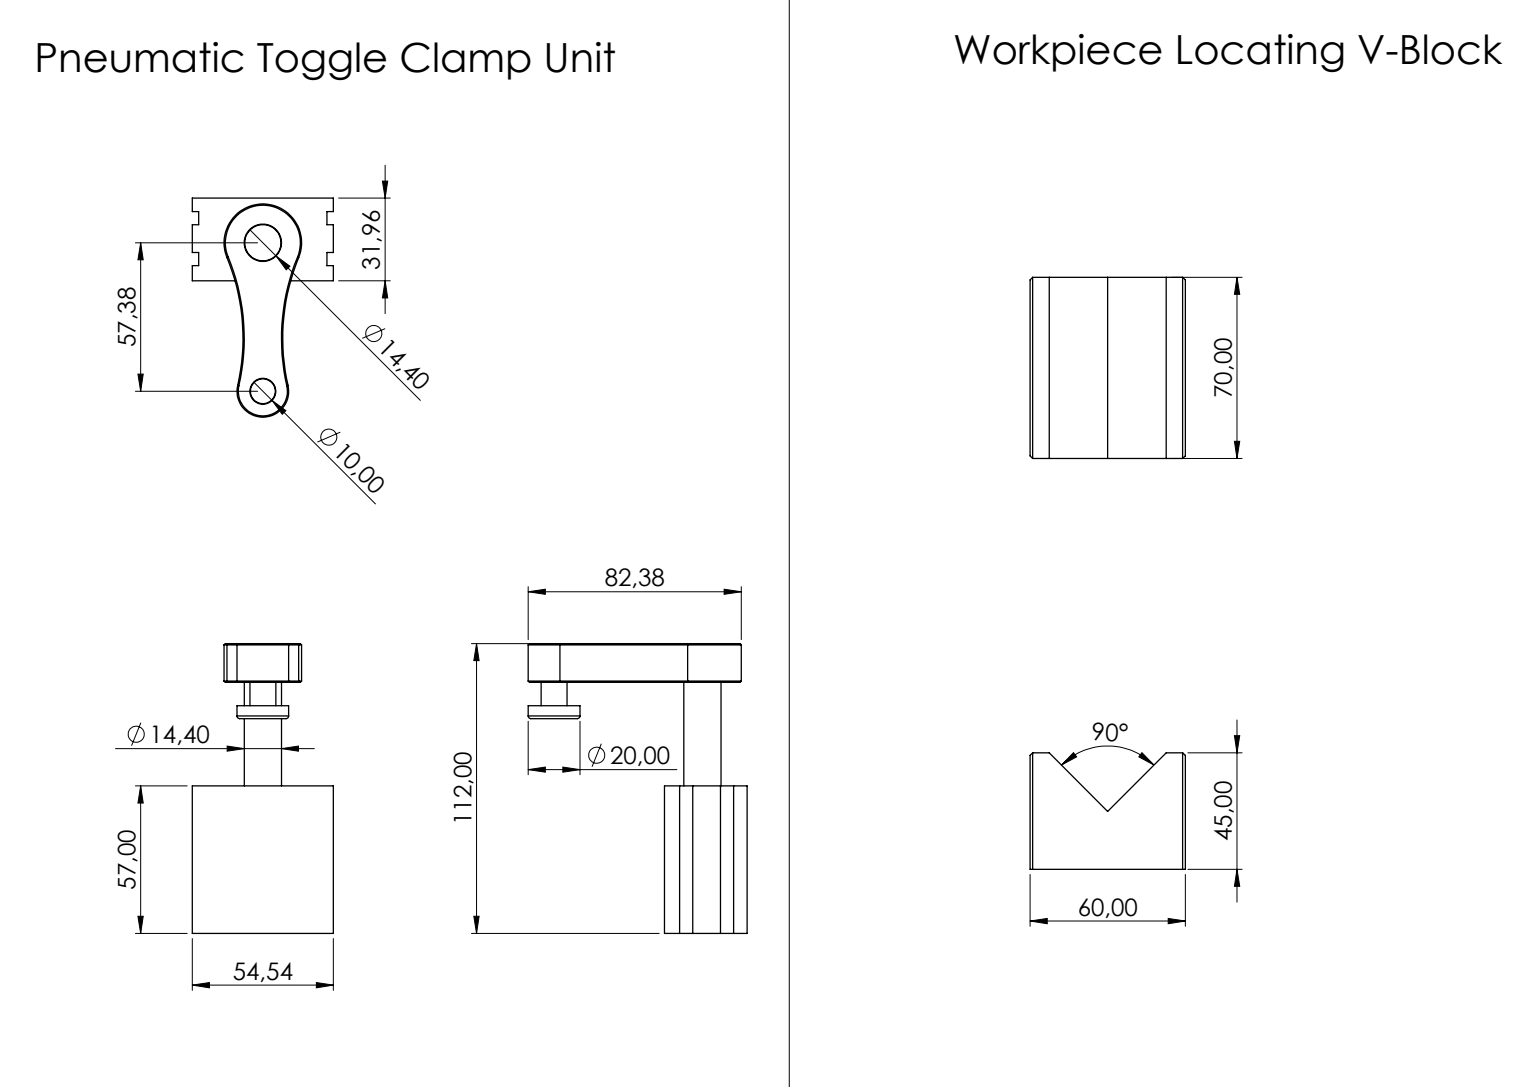
ISO-10303-21;
HEADER;
FILE_DESCRIPTION (('STEP AP214'),
    '1' );
FILE_NAME ('Workpiece Locating V-Block.step',
    '2026-10-07T11:37:37',
    ( '' ),
    ( '' ),
    'SwSTEP 2.0',
    'SolidWorks 2020',
    '' );
FILE_SCHEMA (( 'AUTOMOTIVE_DESIGN' ));
ENDSEC;

DATA;
#31=VECTOR ( 'NONE', #9113, 1000.000000000000000 ) ;
#48=LINE ( 'NONE', #40482, #73685 ) ;
#312=CARTESIAN_POINT ( 'NONE',  ( 29.00000000000003553, 172.0000000000000000, 183.8826257785461280 ) ) ;
#346=EDGE_LOOP ( 'NONE', ( #42852, #56752, #84948, #3553, #65109, #46842, #22187 ) ) ;
#557=EDGE_LOOP ( 'NONE', ( #41449, #70059, #56330, #26549 ) ) ;
#745=ORIENTED_EDGE ( 'NONE', *, *, #84172, .F. ) ;
#885=SHAPE_REPRESENTATION ( 'Workpiece Locating V-Block', ( #50656 ), #34903 ) ;
#1117=FILL_AREA_STYLE ('',( #49240 ) ) ;
#1367=EDGE_LOOP ( 'NONE', ( #36346, #35082, #79316, #26677 ) ) ;
#1388=ADVANCED_FACE ( 'NONE', ( #30270 ), #32030, .F. ) ;
#1574=( LENGTH_UNIT ( ) NAMED_UNIT ( * ) SI_UNIT ( .MILLI., .METRE. ) );
#2105=ORIENTED_EDGE ( 'NONE', *, *, #24082, .F. ) ;
#2350=PLANE ( 'NONE',  #26051 ) ;
#2410=FACE_OUTER_BOUND ( 'NONE', #58762, .T. ) ;
#2579=VECTOR ( 'NONE', #6464, 1000.000000000000000 ) ;
#2820=STYLED_ITEM ( 'NONE', ( #7866 ), #65184 ) ;
#2899=DIRECTION ( 'NONE',  ( 0.000000000000000000, 1.000000000000000000, 0.000000000000000000 ) ) ;
#3553=ORIENTED_EDGE ( 'NONE', *, *, #14732, .F. ) ;
#3670=VECTOR ( 'NONE', #89572, 1000.000000000000000 ) ;
#3713=ORIENTED_EDGE ( 'NONE', *, *, #21319, .F. ) ;
#3849=LINE ( 'NONE', #9776, #78567 ) ;
#4788=LINE ( 'NONE', #5235, #17155 ) ;
#5235=CARTESIAN_POINT ( 'NONE',  ( -28.99999999999997513, 172.0000000000000000, 183.8826257785461280 ) ) ;
#5543=LINE ( 'NONE', #54539, #85490 ) ;
#5568=CARTESIAN_POINT ( 'NONE',  ( -28.99999999999997513, 172.0000000000000000, 183.8826257785461280 ) ) ;
#5571=DIRECTION ( 'NONE',  ( -2.973811673103097665E-16, 0.000000000000000000, -1.000000000000000000 ) ) ;
#5616=AXIS2_PLACEMENT_3D ( 'NONE', #25293, #52962, #18474 ) ;
#5642=DIRECTION ( 'NONE',  ( 1.000000000000000000, 0.000000000000000000, 0.000000000000000000 ) ) ;
#5959=EDGE_CURVE ( 'NONE', #84182, #45804, #3849, .T. ) ;
#6325=ADVANCED_FACE ( 'NONE', ( #2410 ), #72785, .F. ) ;
#6464=DIRECTION ( 'NONE',  ( -0.000000000000000000, -0.000000000000000000, 1.000000000000000000 ) ) ;
#6549=AXIS2_PLACEMENT_3D ( 'NONE', #16158, #31547, #65187 ) ;
#6568=AXIS2_PLACEMENT_3D ( 'NONE', #5568, #33260, #74592 ) ;
#6613=EDGE_CURVE ( 'NONE', #83706, #79712, #41817, .T. ) ;
#6688=LINE ( 'NONE', #62098, #79473 ) ;
#6802=ORIENTED_EDGE ( 'NONE', *, *, #6613, .T. ) ;
#6910=LINE ( 'NONE', #33727, #2579 ) ;
#7127=DIRECTION ( 'NONE',  ( 0.000000000000000000, -1.000000000000000000, 0.000000000000000000 ) ) ;
#7155=CARTESIAN_POINT ( 'NONE',  ( -22.62762465138237644, 172.0000000000000000, 183.8826257785461280 ) ) ;
#7836=DIRECTION ( 'NONE',  ( -2.973811673103097665E-16, -0.000000000000000000, -1.000000000000000000 ) ) ;
#7866=PRESENTATION_STYLE_ASSIGNMENT (( #76915 ) ) ;
#7925=PRESENTATION_STYLE_ASSIGNMENT (( #70153 ) ) ;
#7955=ORIENTED_EDGE ( 'NONE', *, *, #36671, .F. ) ;
#8029=VECTOR ( 'NONE', #67867, 1000.000000000000000 ) ;
#8038=CARTESIAN_POINT ( 'NONE',  ( 29.00000000000001421, 127.0000000000000000, 113.8826257785461280 ) ) ;
#8263=DIRECTION ( 'NONE',  ( 0.000000000000000000, 1.000000000000000000, 0.000000000000000000 ) ) ;
#8323=CARTESIAN_POINT ( 'NONE',  ( -22.62762465138237644, 172.0000000000000000, 183.8826257785461280 ) ) ;
#8780=LINE ( 'NONE', #8323, #31223 ) ;
#9046=VECTOR ( 'NONE', #27312, 1000.000000000000114 ) ;
#9113=DIRECTION ( 'NONE',  ( 1.000000000000000000, 0.000000000000000000, 0.000000000000000000 ) ) ;
#9427=DIRECTION ( 'NONE',  ( 2.973811673103097665E-16, 0.000000000000000000, 1.000000000000000000 ) ) ;
#9776=CARTESIAN_POINT ( 'NONE',  ( -29.99999999999998224, 127.0000000000000000, 114.8826257785461280 ) ) ;
#9798=VERTEX_POINT ( 'NONE', #44981 ) ;
#9823=DIRECTION ( 'NONE',  ( 1.000000000000000000, 0.000000000000000000, -0.000000000000000000 ) ) ;
#10551=DIRECTION ( 'NONE',  ( -0.7071067811865462405, -0.7071067811865489050, 0.000000000000000000 ) ) ;
#10810=CARTESIAN_POINT ( 'NONE',  ( 30.00000000000003553, 172.0000000000000000, 182.8826257785461280 ) ) ;
#10831=DIRECTION ( 'NONE',  ( 2.973811673103097665E-16, -0.000000000000000000, 1.000000000000000000 ) ) ;
#10860=EDGE_CURVE ( 'NONE', #52412, #74795, #6910, .T. ) ;
#10913=EDGE_CURVE ( 'NONE', #57450, #52412, #13729, .T. ) ;
#11030=EDGE_CURVE ( 'NONE', #79712, #48254, #64124, .T. ) ;
#11412=FACE_OUTER_BOUND ( 'NONE', #55786, .T. ) ;
#11674=CARTESIAN_POINT ( 'NONE',  ( 6.938893903907228378E-15, 149.3723753486177088, 183.8826257785461280 ) ) ;
#11676=ORIENTED_EDGE ( 'NONE', *, *, #83356, .F. ) ;
#11927=PLANE ( 'NONE',  #6568 ) ;
#11953=VERTEX_POINT ( 'NONE', #7155 ) ;
#11964=CARTESIAN_POINT ( 'NONE',  ( -29.99999999999998224, 127.0000000000000000, 113.8826257785461280 ) ) ;
#12184=DIRECTION ( 'NONE',  ( -2.973811673103097665E-16, 0.000000000000000000, -1.000000000000000000 ) ) ;
#12403=LINE ( 'NONE', #11964, #52330 ) ;
#12461=LINE ( 'NONE', #40146, #8029 ) ;
#13286=EDGE_CURVE ( 'NONE', #89067, #69114, #54123, .T. ) ;
#13729=LINE ( 'NONE', #55029, #51872 ) ;
#13785=( NAMED_UNIT ( * ) SI_UNIT ( $, .STERADIAN. ) SOLID_ANGLE_UNIT ( ) );
#13831=VECTOR ( 'NONE', #5571, 1000.000000000000000 ) ;
#14314=FACE_OUTER_BOUND ( 'NONE', #346, .T. ) ;
#14555=VECTOR ( 'NONE', #79134, 1000.000000000000000 ) ;
#14616=CARTESIAN_POINT ( 'NONE',  ( 29.00000000000001421, 172.0000000000000000, 113.8826257785461280 ) ) ;
#14639=LINE ( 'NONE', #70495, #89443 ) ;
#14732=EDGE_CURVE ( 'NONE', #74795, #76086, #14639, .T. ) ;
#16124=ORIENTED_EDGE ( 'NONE', *, *, #24370, .T. ) ;
#16158=CARTESIAN_POINT ( 'NONE',  ( 0.000000000000000000, 172.0000000000000000, 0.000000000000000000 ) ) ;
#16735=VECTOR ( 'NONE', #51173, 1000.000000000000114 ) ;
#16836=DIRECTION ( 'NONE',  ( 0.5773502691896258421, -0.5773502691896255090, -0.5773502691896258421 ) ) ;
#17001=EDGE_CURVE ( 'NONE', #64475, #75853, #55572, .T. ) ;
#17006=AXIS2_PLACEMENT_3D ( 'NONE', #48469, #41668, #82607 ) ;
#17124=CARTESIAN_POINT ( 'NONE',  ( -3.686187674308976980, 145.6861876743087691, 113.8826257785461280 ) ) ;
#17155=VECTOR ( 'NONE', #32924, 1000.000000000000114 ) ;
#17401=PRODUCT_DEFINITION_FORMATION_WITH_SPECIFIED_SOURCE ( 'ANY', '', #73550, .NOT_KNOWN. ) ;
#17787=EDGE_LOOP ( 'NONE', ( #23547, #11676, #2105, #23295 ) ) ;
#17821=DIRECTION ( 'NONE',  ( 0.000000000000000000, -1.000000000000000000, 0.000000000000000000 ) ) ;
#18011=LINE ( 'NONE', #51184, #34516 ) ;
#18088=CARTESIAN_POINT ( 'NONE',  ( -29.00000000000002842, 172.0000000000000000, 8.624053851998991955E-15 ) ) ;
#18474=DIRECTION ( 'NONE',  ( -2.973811673103097665E-16, 0.000000000000000000, -1.000000000000000000 ) ) ;
#18531=ORIENTED_EDGE ( 'NONE', *, *, #68420, .T. ) ;
#19066=ORIENTED_EDGE ( 'NONE', *, *, #40506, .T. ) ;
#19070=CARTESIAN_POINT ( 'NONE',  ( -29.99999999999998224, 172.0000000000000000, 113.8826257785461280 ) ) ;
#19265=DIRECTION ( 'NONE',  ( 0.000000000000000000, 0.000000000000000000, 1.000000000000000000 ) ) ;
#19294=CARTESIAN_POINT ( 'NONE',  ( 30.00000000000001776, 172.0000000000000000, 114.8826257785461280 ) ) ;
#19330=CARTESIAN_POINT ( 'NONE',  ( -29.99999999999996092, 172.0000000000000000, 183.8826257785461280 ) ) ;
#19948=CARTESIAN_POINT ( 'NONE',  ( 8.960875259515155733, 209.9608752595157455, 75.92175051903043936 ) ) ;
#19984=ORIENTED_EDGE ( 'NONE', *, *, #82440, .F. ) ;
#19996=VERTEX_POINT ( 'NONE', #59788 ) ;
#20939=DIRECTION ( 'NONE',  ( 0.000000000000000000, 0.000000000000000000, 1.000000000000000000 ) ) ;
#21093=CARTESIAN_POINT ( 'NONE',  ( -28.99999999999997513, 127.0000000000000000, 183.8826257785461280 ) ) ;
#21319=EDGE_CURVE ( 'NONE', #83706, #77060, #35084, .T. ) ;
#21403=EDGE_LOOP ( 'NONE', ( #22104, #78884, #37129, #38666, #745, #52148, #29845 ) ) ;
#21512=FILL_AREA_STYLE_COLOUR ( '', #78446 ) ;
#21966=( NAMED_UNIT ( * ) PLANE_ANGLE_UNIT ( ) SI_UNIT ( $, .RADIAN. ) );
#22048=ORIENTED_EDGE ( 'NONE', *, *, #65025, .F. ) ;
#22104=ORIENTED_EDGE ( 'NONE', *, *, #73838, .F. ) ;
#22187=ORIENTED_EDGE ( 'NONE', *, *, #36671, .T. ) ;
#22916=( NAMED_UNIT ( * ) PLANE_ANGLE_UNIT ( ) SI_UNIT ( $, .RADIAN. ) );
#22948=AXIS2_PLACEMENT_3D ( 'NONE', #23469, #31142, #9823 ) ;
#23079=VERTEX_POINT ( 'NONE', #59557 ) ;
#23160=DIRECTION ( 'NONE',  ( 0.7071067811865471286, 0.7071067811865479058, -2.102802400022911660E-16 ) ) ;
#23172=APPLICATION_CONTEXT ( 'automotive_design' ) ;
#23295=ORIENTED_EDGE ( 'NONE', *, *, #67596, .F. ) ;
#23469=CARTESIAN_POINT ( 'NONE',  ( -29.99999999999998224, 172.0000000000000000, 113.8826257785461280 ) ) ;
#23547=ORIENTED_EDGE ( 'NONE', *, *, #69307, .T. ) ;
#23641=LINE ( 'NONE', #64073, #31 ) ;
#23663=CARTESIAN_POINT ( 'NONE',  ( 29.66666666666670338, 171.3333333333333428, 183.2159591118794708 ) ) ;
#23991=ORIENTED_EDGE ( 'NONE', *, *, #81901, .T. ) ;
#24082=EDGE_CURVE ( 'NONE', #30852, #77060, #47509, .T. ) ;
#24230=CLOSED_SHELL ( 'NONE', ( #24261, #43904, #1388, #88028, #36060, #30256, #37908, #43206, #6325, #30529, #70524, #64945, #59102, #51035, #72629 ) ) ;
#24261=ADVANCED_FACE ( 'NONE', ( #57473 ), #85213, .T. ) ;
#24370=EDGE_CURVE ( 'NONE', #19996, #83706, #55097, .T. ) ;
#24445=ORIENTED_EDGE ( 'NONE', *, *, #24370, .F. ) ;
#25293=CARTESIAN_POINT ( 'NONE',  ( -29.99999999999998224, 172.0000000000000000, 113.8826257785461280 ) ) ;
#25787=CARTESIAN_POINT ( 'NONE',  ( -29.99999999999998224, 171.0000000000000000, 114.8826257785461280 ) ) ;
#26010=ORIENTED_EDGE ( 'NONE', *, *, #13286, .F. ) ;
#26051=AXIS2_PLACEMENT_3D ( 'NONE', #85031, #86361, #50477 ) ;
#26383=AXIS2_PLACEMENT_3D ( 'NONE', #86472, #2899, #84692 ) ;
#26549=ORIENTED_EDGE ( 'NONE', *, *, #86670, .T. ) ;
#26677=ORIENTED_EDGE ( 'NONE', *, *, #87182, .F. ) ;
#26944=CARTESIAN_POINT ( 'NONE',  ( 30.00000000000001776, 127.0000000000000000, 113.8826257785461280 ) ) ;
#27088=ORIENTED_EDGE ( 'NONE', *, *, #73838, .T. ) ;
#27312=DIRECTION ( 'NONE',  ( -0.7071067811865474617, -0.000000000000000000, 0.7071067811865474617 ) ) ;
#27583=DIRECTION ( 'NONE',  ( 0.5773502691896260641, -0.5773502691896252870, 0.5773502691896260641 ) ) ;
#28322=CARTESIAN_POINT ( 'NONE',  ( 22.62762465138250789, 172.0000000000000000, 0.000000000000000000 ) ) ;
#28765=( NAMED_UNIT ( * ) PLANE_ANGLE_UNIT ( ) SI_UNIT ( $, .RADIAN. ) );
#29275=( NAMED_UNIT ( * ) SI_UNIT ( $, .STERADIAN. ) SOLID_ANGLE_UNIT ( ) );
#29845=ORIENTED_EDGE ( 'NONE', *, *, #80138, .T. ) ;
#29936=ORIENTED_EDGE ( 'NONE', *, *, #10860, .F. ) ;
#30221=CARTESIAN_POINT ( 'NONE',  ( -28.99999999999997513, 127.0000000000000000, 183.8826257785461280 ) ) ;
#30256=ADVANCED_FACE ( 'NONE', ( #57851 ), #58728, .T. ) ;
#30270=FACE_OUTER_BOUND ( 'NONE', #21403, .T. ) ;
#30529=ADVANCED_FACE ( 'NONE', ( #52126 ), #32148, .F. ) ;
#30852=VERTEX_POINT ( 'NONE', #8038 ) ;
#31016=ORIENTED_EDGE ( 'NONE', *, *, #5959, .T. ) ;
#31142=DIRECTION ( 'NONE',  ( 0.000000000000000000, 0.000000000000000000, 1.000000000000000000 ) ) ;
#31223=VECTOR ( 'NONE', #36021, 1000.000000000000000 ) ;
#31252=DIRECTION ( 'NONE',  ( 0.000000000000000000, -1.000000000000000000, 0.000000000000000000 ) ) ;
#31382=VECTOR ( 'NONE', #44907, 1000.000000000000000 ) ;
#31528=VECTOR ( 'NONE', #8263, 1000.000000000000000 ) ;
#31547=DIRECTION ( 'NONE',  ( 0.000000000000000000, 1.000000000000000000, 0.000000000000000000 ) ) ;
#32030=PLANE ( 'NONE',  #22948 ) ;
#32037=CARTESIAN_POINT ( 'NONE',  ( 22.62762465138245460, 171.9999999999999716, 96.88262577854611379 ) ) ;
#32104=FACE_OUTER_BOUND ( 'NONE', #557, .T. ) ;
#32148=PLANE ( 'NONE',  #53910 ) ;
#32287=CARTESIAN_POINT ( 'NONE',  ( -29.99999999999998224, 127.0000000000000000, 113.8826257785461280 ) ) ;
#32754=ORIENTED_EDGE ( 'NONE', *, *, #35969, .T. ) ;
#32809=ORIENTED_EDGE ( 'NONE', *, *, #80138, .F. ) ;
#32839=DIRECTION ( 'NONE',  ( 2.973811673103097665E-16, 0.000000000000000000, 1.000000000000000000 ) ) ;
#32924=DIRECTION ( 'NONE',  ( 0.5773502691896201799, 0.5773502691896286176, 0.5773502691896283956 ) ) ;
#32943=LINE ( 'NONE', #19330, #61992 ) ;
#32954=VECTOR ( 'NONE', #9427, 1000.000000000000000 ) ;
#32997=DIRECTION ( 'NONE',  ( 0.7071067811865474617, -0.000000000000000000, 0.7071067811865474617 ) ) ;
#33260=DIRECTION ( 'NONE',  ( 0.7071067811865524577, 0.000000000000000000, -0.7071067811865425767 ) ) ;
#33450=CARTESIAN_POINT ( 'NONE',  ( 29.00000000000001421, 127.0000000000000000, 113.8826257785461280 ) ) ;
#33727=CARTESIAN_POINT ( 'NONE',  ( 6.938893903907228378E-15, 149.3723753486177088, 96.88262577854611379 ) ) ;
#33846=CARTESIAN_POINT ( 'NONE',  ( -29.99999999999996092, 172.0000000000000000, 183.8826257785461280 ) ) ;
#34516=VECTOR ( 'NONE', #52064, 1000.000000000000000 ) ;
#34528=ORIENTED_EDGE ( 'NONE', *, *, #45193, .F. ) ;
#34529=EDGE_CURVE ( 'NONE', #88820, #46473, #84364, .T. ) ;
#34688=CARTESIAN_POINT ( 'NONE',  ( -22.62762465138237999, 172.0000000000000000, 113.8826257785461280 ) ) ;
#34903=( GEOMETRIC_REPRESENTATION_CONTEXT ( 3 ) GLOBAL_UNCERTAINTY_ASSIGNED_CONTEXT ( ( #39922 ) ) GLOBAL_UNIT_ASSIGNED_CONTEXT ( ( #70093, #28765, #13785 ) ) REPRESENTATION_CONTEXT ( 'NONE', 'WORKASPACE' ) );
#35082=ORIENTED_EDGE ( 'NONE', *, *, #34529, .T. ) ;
#35084=LINE ( 'NONE', #26944, #82856 ) ;
#35502=DIRECTION ( 'NONE',  ( 0.7071067811865507924, 0.7071067811865441310, -0.000000000000000000 ) ) ;
#35729=DIRECTION ( 'NONE',  ( 2.973811673103097665E-16, 0.000000000000000000, 1.000000000000000000 ) ) ;
#35737=COLOUR_RGB ( '', 0.40784314, 0.44705882, 0.49803922) ;
#35969=EDGE_CURVE ( 'NONE', #76086, #48254, #32943, .T. ) ;
#36021=DIRECTION ( 'NONE',  ( 0.7071067811865489050, -0.7071067811865462405, 0.000000000000000000 ) ) ;
#36060=ADVANCED_FACE ( 'NONE', ( #14314 ), #47900, .F. ) ;
#36346=ORIENTED_EDGE ( 'NONE', *, *, #84172, .T. ) ;
#36582=LINE ( 'NONE', #57900, #75628 ) ;
#36671=EDGE_CURVE ( 'NONE', #46473, #64475, #58536, .T. ) ;
#37009=ORIENTED_EDGE ( 'NONE', *, *, #72553, .F. ) ;
#37070=VECTOR ( 'NONE', #59938, 1000.000000000000000 ) ;
#37129=ORIENTED_EDGE ( 'NONE', *, *, #72553, .T. ) ;
#37212=CARTESIAN_POINT ( 'NONE',  ( 28.99999999999998224, 172.0000000000000000, -8.624053851998977755E-15 ) ) ;
#37609=AXIS2_PLACEMENT_3D ( 'NONE', #32037, #42421, #69708 ) ;
#37786=DIRECTION ( 'NONE',  ( 0.7071067811865524577, 0.000000000000000000, 0.7071067811865425767 ) ) ;
#37897=ORIENTED_EDGE ( 'NONE', *, *, #6613, .F. ) ;
#37908=ADVANCED_FACE ( 'NONE', ( #83481 ), #89409, .F. ) ;
#37949=ORIENTED_EDGE ( 'NONE', *, *, #17001, .F. ) ;
#38011=AXIS2_PLACEMENT_3D ( 'NONE', #80058, #10551, #58685 ) ;
#38224=CARTESIAN_POINT ( 'NONE',  ( -29.99999999999998224, 172.0000000000000000, 114.8826257785461280 ) ) ;
#38242=ORIENTED_EDGE ( 'NONE', *, *, #10913, .F. ) ;
#38257=CARTESIAN_POINT ( 'NONE',  ( -29.99999999999996092, 127.0000000000000000, 182.8826257785461280 ) ) ;
#38666=ORIENTED_EDGE ( 'NONE', *, *, #82015, .T. ) ;
#38883=ORIENTED_EDGE ( 'NONE', *, *, #69307, .F. ) ;
#39494=SHAPE_DEFINITION_REPRESENTATION ( #45226, #885 ) ;
#39697=CARTESIAN_POINT ( 'NONE',  ( 30.00000000000003553, 172.0000000000000000, 182.8826257785461280 ) ) ;
#39922=UNCERTAINTY_MEASURE_WITH_UNIT (LENGTH_MEASURE( 1.000000000000000082E-05 ), #70093, 'distance_accuracy_value', 'NONE');
#39930=VECTOR ( 'NONE', #61933, 1000.000000000000000 ) ;
#39967=APPLICATION_CONTEXT ( 'automotive_design' ) ;
#39970=VECTOR ( 'NONE', #16836, 1000.000000000000114 ) ;
#40037=FACE_OUTER_BOUND ( 'NONE', #17787, .T. ) ;
#40146=CARTESIAN_POINT ( 'NONE',  ( -28.99999999999999289, 172.0000000000000000, 113.8826257785461280 ) ) ;
#40186=FACE_OUTER_BOUND ( 'NONE', #55339, .T. ) ;
#40482=CARTESIAN_POINT ( 'NONE',  ( -22.62762465138237999, 172.0000000000000000, 0.000000000000000000 ) ) ;
#40506=EDGE_CURVE ( 'NONE', #69114, #88820, #48964, .T. ) ;
#41086=PLANE ( 'NONE',  #37609 ) ;
#41449=ORIENTED_EDGE ( 'NONE', *, *, #13286, .T. ) ;
#41471=( NAMED_UNIT ( * ) SI_UNIT ( $, .STERADIAN. ) SOLID_ANGLE_UNIT ( ) );
#41668=DIRECTION ( 'NONE',  ( 0.000000000000000000, 1.000000000000000000, 0.000000000000000000 ) ) ;
#41817=LINE ( 'NONE', #42273, #9046 ) ;
#42273=CARTESIAN_POINT ( 'NONE',  ( 30.00000000000003553, 127.0000000000000000, 182.8826257785461280 ) ) ;
#42421=DIRECTION ( 'NONE',  ( 0.7071067811865442421, -0.7071067811865509034, 0.000000000000000000 ) ) ;
#42429=SURFACE_STYLE_FILL_AREA ( #1117 ) ;
#42658=EDGE_LOOP ( 'NONE', ( #37949, #7955, #63053, #86622 ) ) ;
#42766=ORIENTED_EDGE ( 'NONE', *, *, #11030, .F. ) ;
#42771=VECTOR ( 'NONE', #32997, 1000.000000000000114 ) ;
#42852=ORIENTED_EDGE ( 'NONE', *, *, #65025, .T. ) ;
#43206=ADVANCED_FACE ( 'NONE', ( #40186 ), #41086, .F. ) ;
#43368=AXIS2_PLACEMENT_3D ( 'NONE', #74123, #66854, #53189 ) ;
#43904=ADVANCED_FACE ( 'NONE', ( #57747 ), #2350, .F. ) ;
#44352=VECTOR ( 'NONE', #35729, 1000.000000000000000 ) ;
#44907=DIRECTION ( 'NONE',  ( 0.000000000000000000, -1.000000000000000000, 0.000000000000000000 ) ) ;
#44981=CARTESIAN_POINT ( 'NONE',  ( 30.00000000000001776, 171.0000000000000000, 114.8826257785461280 ) ) ;
#45193=EDGE_CURVE ( 'NONE', #84182, #75853, #12403, .T. ) ;
#45226=PRODUCT_DEFINITION_SHAPE ( 'NONE', 'NONE',  #61043 ) ;
#45804=VERTEX_POINT ( 'NONE', #64527 ) ;
#45941=CARTESIAN_POINT ( 'NONE',  ( -29.99999999999998224, 172.0000000000000000, 114.8826257785461280 ) ) ;
#45959=CARTESIAN_POINT ( 'NONE',  ( 30.00000000000003553, 127.0000000000000000, 182.8826257785461280 ) ) ;
#46172=CARTESIAN_POINT ( 'NONE',  ( 6.938893903907228378E-15, 149.3723753486177088, 113.8826257785461280 ) ) ;
#46389=PLANE ( 'NONE',  #43368 ) ;
#46473=VERTEX_POINT ( 'NONE', #59809 ) ;
#46526=DIRECTION ( 'NONE',  ( 0.000000000000000000, 1.000000000000000000, 0.000000000000000000 ) ) ;
#46679=PLANE ( 'NONE',  #47457 ) ;
#46754=LINE ( 'NONE', #19070, #37070 ) ;
#46841=LINE ( 'NONE', #45941, #70470 ) ;
#46842=ORIENTED_EDGE ( 'NONE', *, *, #89398, .F. ) ;
#47457=AXIS2_PLACEMENT_3D ( 'NONE', #18088, #74409, #12184 ) ;
#47509=LINE ( 'NONE', #33450, #42771 ) ;
#47900=PLANE ( 'NONE',  #75036 ) ;
#47984=CARTESIAN_POINT ( 'NONE',  ( 29.00000000000001421, 172.0000000000000000, 113.8826257785461280 ) ) ;
#47986=EDGE_LOOP ( 'NONE', ( #32754, #63928, #27088, #65250 ) ) ;
#48254=VERTEX_POINT ( 'NONE', #312 ) ;
#48469=CARTESIAN_POINT ( 'NONE',  ( 0.000000000000000000, 127.0000000000000000, 0.000000000000000000 ) ) ;
#48964=LINE ( 'NONE', #19948, #77879 ) ;
#49063=EDGE_LOOP ( 'NONE', ( #68351, #71266, #52444, #16124 ) ) ;
#49181=SURFACE_STYLE_FILL_AREA ( #83286 ) ;
#49240=FILL_AREA_STYLE_COLOUR ( '', #35737 ) ;
#49407=AXIS2_PLACEMENT_3D ( 'NONE', #38224, #37786, #86830 ) ;
#50041=MANIFOLD_SOLID_BREP ( 'Stock-BR-Y-104-1', #24230 ) ;
#50477=DIRECTION ( 'NONE',  ( 2.973811673103097665E-16, 0.000000000000000000, 1.000000000000000000 ) ) ;
#50656=AXIS2_PLACEMENT_3D ( 'NONE', #89656, #19265, #5642 ) ;
#51035=ADVANCED_FACE ( 'NONE', ( #54371 ), #46679, .T. ) ;
#51173=DIRECTION ( 'NONE',  ( 0.7071067811865507924, 0.7071067811865441310, -0.000000000000000000 ) ) ;
#51184=CARTESIAN_POINT ( 'NONE',  ( -29.99999999999996092, 172.0000000000000000, 182.8826257785461280 ) ) ;
#51691=DIRECTION ( 'NONE',  ( -0.7071067811865475727, -0.000000000000000000, -0.7071067811865475727 ) ) ;
#51872=VECTOR ( 'NONE', #88261, 1000.000000000000000 ) ;
#52064=DIRECTION ( 'NONE',  ( 0.000000000000000000, 1.000000000000000000, 0.000000000000000000 ) ) ;
#52126=FACE_OUTER_BOUND ( 'NONE', #64103, .T. ) ;
#52142=PLANE ( 'NONE',  #70913 ) ;
#52148=ORIENTED_EDGE ( 'NONE', *, *, #10913, .T. ) ;
#52330=VECTOR ( 'NONE', #32839, 1000.000000000000000 ) ;
#52412=VERTEX_POINT ( 'NONE', #46172 ) ;
#52444=ORIENTED_EDGE ( 'NONE', *, *, #80998, .T. ) ;
#52962=DIRECTION ( 'NONE',  ( 1.000000000000000000, 0.000000000000000000, -2.973811673103097665E-16 ) ) ;
#53143=MECHANICAL_DESIGN_GEOMETRIC_PRESENTATION_REPRESENTATION('',(#83612),#77840);
#53189=DIRECTION ( 'NONE',  ( 0.000000000000000000, -1.000000000000000000, 0.000000000000000000 ) ) ;
#53897=ORIENTED_EDGE ( 'NONE', *, *, #17001, .T. ) ;
#53910=AXIS2_PLACEMENT_3D ( 'NONE', #10810, #51691, #31252 ) ;
#54123=LINE ( 'NONE', #88249, #13831 ) ;
#54371=FACE_OUTER_BOUND ( 'NONE', #84498, .T. ) ;
#54539=CARTESIAN_POINT ( 'NONE',  ( -29.99999999999996092, 127.0000000000000000, 183.8826257785461280 ) ) ;
#54789=VECTOR ( 'NONE', #7127, 1000.000000000000000 ) ;
#55029=CARTESIAN_POINT ( 'NONE',  ( -26.31381232569119533, 175.6861876743088260, 113.8826257785461280 ) ) ;
#55097=LINE ( 'NONE', #39697, #39930 ) ;
#55114=LINE ( 'NONE', #28322, #82448 ) ;
#55339=EDGE_LOOP ( 'NONE', ( #80154, #86313, #82824, #32809 ) ) ;
#55572=LINE ( 'NONE', #21093, #80267 ) ;
#55786=EDGE_LOOP ( 'NONE', ( #19066, #81340, #57636, #19984 ) ) ;
#56330=ORIENTED_EDGE ( 'NONE', *, *, #45193, .T. ) ;
#56630=VERTEX_POINT ( 'NONE', #60935 ) ;
#56752=ORIENTED_EDGE ( 'NONE', *, *, #11030, .T. ) ;
#56904=SURFACE_SIDE_STYLE ('',( #49181 ) ) ;
#57108=CARTESIAN_POINT ( 'NONE',  ( 30.00000000000003553, 171.0000000000000000, 183.8826257785461280 ) ) ;
#57450=VERTEX_POINT ( 'NONE', #34688 ) ;
#57473=FACE_OUTER_BOUND ( 'NONE', #47986, .T. ) ;
#57636=ORIENTED_EDGE ( 'NONE', *, *, #5959, .F. ) ;
#57747=FACE_OUTER_BOUND ( 'NONE', #49063, .T. ) ;
#57851=FACE_OUTER_BOUND ( 'NONE', #1367, .T. ) ;
#57900=CARTESIAN_POINT ( 'NONE',  ( -29.99999999999998224, 172.0000000000000000, 113.8826257785461280 ) ) ;
#58536=LINE ( 'NONE', #64476, #31382 ) ;
#58573=ORIENTED_EDGE ( 'NONE', *, *, #83854, .F. ) ;
#58685=DIRECTION ( 'NONE',  ( 0.7071067811865489050, -0.7071067811865462405, 0.000000000000000000 ) ) ;
#58728=PLANE ( 'NONE',  #26383 ) ;
#58762=EDGE_LOOP ( 'NONE', ( #79445, #23991, #29936, #38242 ) ) ;
#59102=ADVANCED_FACE ( 'NONE', ( #61401 ), #11927, .F. ) ;
#59321=ORIENTED_EDGE ( 'NONE', *, *, #34529, .F. ) ;
#59557=CARTESIAN_POINT ( 'NONE',  ( 22.62762465138245460, 171.9999999999999716, 113.8826257785461280 ) ) ;
#59788=CARTESIAN_POINT ( 'NONE',  ( 30.00000000000003553, 171.0000000000000000, 182.8826257785461280 ) ) ;
#59799=PLANE ( 'NONE',  #5616 ) ;
#59809=CARTESIAN_POINT ( 'NONE',  ( -28.99999999999997513, 172.0000000000000000, 183.8826257785461280 ) ) ;
#59938=DIRECTION ( 'NONE',  ( -1.000000000000000000, -0.000000000000000000, -0.000000000000000000 ) ) ;
#60935=CARTESIAN_POINT ( 'NONE',  ( 29.00000000000001421, 172.0000000000000000, 113.8826257785461280 ) ) ;
#61043=PRODUCT_DEFINITION ( 'UNKNOWN', '', #17401, #89895 ) ;
#61401=FACE_OUTER_BOUND ( 'NONE', #42658, .T. ) ;
#61933=DIRECTION ( 'NONE',  ( 0.000000000000000000, -1.000000000000000000, 0.000000000000000000 ) ) ;
#61988=EDGE_CURVE ( 'NONE', #76086, #23079, #55114, .T. ) ;
#61992=VECTOR ( 'NONE', #80227, 1000.000000000000000 ) ;
#62028=ORIENTED_EDGE ( 'NONE', *, *, #80998, .F. ) ;
#62098=CARTESIAN_POINT ( 'NONE',  ( -8.960875259515413305, 209.9608752595154044, 75.92175051903070937 ) ) ;
#63053=ORIENTED_EDGE ( 'NONE', *, *, #68420, .F. ) ;
#63280=( LENGTH_UNIT ( ) NAMED_UNIT ( * ) SI_UNIT ( .MILLI., .METRE. ) );
#63653=LINE ( 'NONE', #14616, #3670 ) ;
#63928=ORIENTED_EDGE ( 'NONE', *, *, #83854, .T. ) ;
#64073=CARTESIAN_POINT ( 'NONE',  ( -29.99999999999996092, 172.0000000000000000, 183.8826257785461280 ) ) ;
#64103=EDGE_LOOP ( 'NONE', ( #37897, #24445, #84483, #42766 ) ) ;
#64124=LINE ( 'NONE', #69593, #31528 ) ;
#64475=VERTEX_POINT ( 'NONE', #30221 ) ;
#64476=CARTESIAN_POINT ( 'NONE',  ( -28.99999999999997513, 172.0000000000000000, 183.8826257785461280 ) ) ;
#64527=CARTESIAN_POINT ( 'NONE',  ( -28.99999999999999289, 127.0000000000000000, 113.8826257785461280 ) ) ;
#64945=ADVANCED_FACE ( 'NONE', ( #40037 ), #46389, .F. ) ;
#65025=EDGE_CURVE ( 'NONE', #64475, #79712, #5543, .T. ) ;
#65109=ORIENTED_EDGE ( 'NONE', *, *, #81901, .F. ) ;
#65184=ADVANCED_BREP_SHAPE_REPRESENTATION ( '', ( #50041, #50656 ), #34903 ) ;
#65187=DIRECTION ( 'NONE',  ( 0.000000000000000000, -0.000000000000000000, 1.000000000000000000 ) ) ;
#65250=ORIENTED_EDGE ( 'NONE', *, *, #61988, .F. ) ;
#66854=DIRECTION ( 'NONE',  ( -0.7071067811865475727, 0.000000000000000000, 0.7071067811865475727 ) ) ;
#67140=DIRECTION ( 'NONE',  ( -0.7071067811865426878, 0.000000000000000000, -0.7071067811865524577 ) ) ;
#67596=EDGE_CURVE ( 'NONE', #56630, #30852, #68905, .T. ) ;
#67867=DIRECTION ( 'NONE',  ( -0.000000000000000000, 1.000000000000000000, 0.000000000000000000 ) ) ;
#68351=ORIENTED_EDGE ( 'NONE', *, *, #21319, .T. ) ;
#68377=DIRECTION ( 'NONE',  ( 0.000000000000000000, 0.000000000000000000, -1.000000000000000000 ) ) ;
#68420=EDGE_CURVE ( 'NONE', #89067, #46473, #4788, .T. ) ;
#68905=LINE ( 'NONE', #47984, #54789 ) ;
#69102=VECTOR ( 'NONE', #46526, 1000.000000000000000 ) ;
#69114=VERTEX_POINT ( 'NONE', #25787 ) ;
#69202=SHAPE_REPRESENTATION_RELATIONSHIP ( 'NONE' , 'NONE' ,  #885, #65184 ) ;
#69307=EDGE_CURVE ( 'NONE', #56630, #9798, #6688, .T. ) ;
#69593=CARTESIAN_POINT ( 'NONE',  ( 29.00000000000003553, 172.0000000000000000, 183.8826257785461280 ) ) ;
#69708=DIRECTION ( 'NONE',  ( 0.7071067811865507924, 0.7071067811865441310, 0.000000000000000000 ) ) ;
#70059=ORIENTED_EDGE ( 'NONE', *, *, #82440, .T. ) ;
#70093=( LENGTH_UNIT ( ) NAMED_UNIT ( * ) SI_UNIT ( .MILLI., .METRE. ) );
#70153=SURFACE_STYLE_USAGE ( .BOTH. , #76977 ) ;
#70162=DIRECTION ( 'NONE',  ( -1.000000000000000000, 0.000000000000000000, -0.000000000000000000 ) ) ;
#70470=VECTOR ( 'NONE', #17821, 1000.000000000000000 ) ;
#70495=CARTESIAN_POINT ( 'NONE',  ( 22.62762465138245460, 171.9999999999999716, 183.8826257785461280 ) ) ;
#70524=ADVANCED_FACE ( 'NONE', ( #71736 ), #52142, .T. ) ;
#70530=EDGE_LOOP ( 'NONE', ( #37009, #74503, #3713, #6802, #22048, #53897, #34528, #31016 ) ) ;
#70913=AXIS2_PLACEMENT_3D ( 'NONE', #37212, #23160, #10831 ) ;
#71266=ORIENTED_EDGE ( 'NONE', *, *, #83356, .T. ) ;
#71736=FACE_OUTER_BOUND ( 'NONE', #73748, .T. ) ;
#71740=CARTESIAN_POINT ( 'NONE',  ( 22.62762465138245460, 171.9999999999999716, 183.8826257785461280 ) ) ;
#71906=CARTESIAN_POINT ( 'NONE',  ( -28.99999999999999289, 172.0000000000000000, 113.8826257785461280 ) ) ;
#72553=EDGE_CURVE ( 'NONE', #30852, #45804, #79581, .T. ) ;
#72629=ADVANCED_FACE ( 'NONE', ( #11412 ), #86384, .F. ) ;
#72785=PLANE ( 'NONE',  #38011 ) ;
#73550=PRODUCT ( 'Workpiece Locating V-Block', 'Workpiece Locating V-Block', '', ( #80852 ) ) ;
#73685=VECTOR ( 'NONE', #20939, 1000.000000000000000 ) ;
#73748=EDGE_LOOP ( 'NONE', ( #83519, #62028, #38883, #58573 ) ) ;
#73838=EDGE_CURVE ( 'NONE', #56630, #23079, #36582, .T. ) ;
#74123=CARTESIAN_POINT ( 'NONE',  ( 29.00000000000001421, 172.0000000000000000, 113.8826257785461280 ) ) ;
#74409=DIRECTION ( 'NONE',  ( -0.7071067811865526798, 0.7071067811865423547, 2.102802400022928177E-16 ) ) ;
#74459=UNCERTAINTY_MEASURE_WITH_UNIT (LENGTH_MEASURE( 1.000000000000000082E-05 ), #1574, 'distance_accuracy_value', 'NONE');
#74503=ORIENTED_EDGE ( 'NONE', *, *, #24082, .T. ) ;
#74592=DIRECTION ( 'NONE',  ( 0.000000000000000000, -1.000000000000000000, 0.000000000000000000 ) ) ;
#74701=LINE ( 'NONE', #19294, #69102 ) ;
#74795=VERTEX_POINT ( 'NONE', #11674 ) ;
#75036=AXIS2_PLACEMENT_3D ( 'NONE', #33846, #68377, #70162 ) ;
#75474=DIRECTION ( 'NONE',  ( 1.000000000000000000, 0.000000000000000000, 0.000000000000000000 ) ) ;
#75504=MECHANICAL_DESIGN_GEOMETRIC_PRESENTATION_REPRESENTATION('',(#2820),#85704);
#75628=VECTOR ( 'NONE', #81393, 1000.000000000000000 ) ;
#75853=VERTEX_POINT ( 'NONE', #38257 ) ;
#76086=VERTEX_POINT ( 'NONE', #71740 ) ;
#76703=DIRECTION ( 'NONE',  ( 0.5773502691896202910, 0.5773502691896288397, -0.5773502691896282846 ) ) ;
#76915=SURFACE_STYLE_USAGE ( .BOTH. , #56904 ) ;
#76977=SURFACE_SIDE_STYLE ('',( #42429 ) ) ;
#77060=VERTEX_POINT ( 'NONE', #84745 ) ;
#77840=( GEOMETRIC_REPRESENTATION_CONTEXT ( 3 ) GLOBAL_UNCERTAINTY_ASSIGNED_CONTEXT ( ( #74459 ) ) GLOBAL_UNIT_ASSIGNED_CONTEXT ( ( #1574, #22916, #29275 ) ) REPRESENTATION_CONTEXT ( 'NONE', 'WORKASPACE' ) );
#77879=VECTOR ( 'NONE', #76703, 1000.000000000000114 ) ;
#78037=LINE ( 'NONE', #57108, #32954 ) ;
#78446=COLOUR_RGB ( '', 0.40784314, 0.44705882, 0.49803922) ;
#78567=VECTOR ( 'NONE', #79281, 1000.000000000000000 ) ;
#78884=ORIENTED_EDGE ( 'NONE', *, *, #67596, .T. ) ;
#79134=DIRECTION ( 'NONE',  ( -1.000000000000000000, -0.000000000000000000, -0.000000000000000000 ) ) ;
#79218=CARTESIAN_POINT ( 'NONE',  ( -28.99999999999997513, 172.0000000000000000, 183.8826257785461280 ) ) ;
#79281=DIRECTION ( 'NONE',  ( 0.7071067811865426878, -0.000000000000000000, -0.7071067811865524577 ) ) ;
#79316=ORIENTED_EDGE ( 'NONE', *, *, #89398, .T. ) ;
#79445=ORIENTED_EDGE ( 'NONE', *, *, #87182, .T. ) ;
#79473=VECTOR ( 'NONE', #27583, 1000.000000000000000 ) ;
#79581=LINE ( 'NONE', #32287, #14555 ) ;
#79712=VERTEX_POINT ( 'NONE', #86996 ) ;
#79918=CARTESIAN_POINT ( 'NONE',  ( -29.99999999999996092, 171.0000000000000000, 182.8826257785461280 ) ) ;
#80058=CARTESIAN_POINT ( 'NONE',  ( -22.62762465138237644, 172.0000000000000000, 96.88262577854611379 ) ) ;
#80138=EDGE_CURVE ( 'NONE', #52412, #23079, #87058, .T. ) ;
#80154=ORIENTED_EDGE ( 'NONE', *, *, #10860, .T. ) ;
#80227=DIRECTION ( 'NONE',  ( 1.000000000000000000, 0.000000000000000000, 0.000000000000000000 ) ) ;
#80267=VECTOR ( 'NONE', #67140, 1000.000000000000000 ) ;
#80852=PRODUCT_CONTEXT ( 'NONE', #39967, 'mechanical' ) ;
#80998=EDGE_CURVE ( 'NONE', #9798, #19996, #78037, .T. ) ;
#81035=ORIENTED_EDGE ( 'NONE', *, *, #40506, .F. ) ;
#81326=CARTESIAN_POINT ( 'NONE',  ( -29.99999999999998224, 127.0000000000000000, 114.8826257785461280 ) ) ;
#81340=ORIENTED_EDGE ( 'NONE', *, *, #82015, .F. ) ;
#81393=DIRECTION ( 'NONE',  ( -1.000000000000000000, -0.000000000000000000, -0.000000000000000000 ) ) ;
#81901=EDGE_CURVE ( 'NONE', #11953, #74795, #8780, .T. ) ;
#82015=EDGE_CURVE ( 'NONE', #45804, #88820, #12461, .T. ) ;
#82440=EDGE_CURVE ( 'NONE', #69114, #84182, #46841, .T. ) ;
#82448=VECTOR ( 'NONE', #82878, 1000.000000000000000 ) ;
#82607=DIRECTION ( 'NONE',  ( 0.000000000000000000, -0.000000000000000000, 1.000000000000000000 ) ) ;
#82743=EDGE_CURVE ( 'NONE', #48254, #19996, #85892, .T. ) ;
#82824=ORIENTED_EDGE ( 'NONE', *, *, #61988, .T. ) ;
#82856=VECTOR ( 'NONE', #7836, 1000.000000000000000 ) ;
#82878=DIRECTION ( 'NONE',  ( 0.000000000000000000, 0.000000000000000000, -1.000000000000000000 ) ) ;
#83286=FILL_AREA_STYLE ('',( #21512 ) ) ;
#83356=EDGE_CURVE ( 'NONE', #77060, #9798, #74701, .T. ) ;
#83481=FACE_OUTER_BOUND ( 'NONE', #70530, .T. ) ;
#83519=ORIENTED_EDGE ( 'NONE', *, *, #82743, .T. ) ;
#83612=STYLED_ITEM ( 'NONE', ( #7925 ), #50041 ) ;
#83706=VERTEX_POINT ( 'NONE', #45959 ) ;
#83854=EDGE_CURVE ( 'NONE', #48254, #56630, #63653, .T. ) ;
#84172=EDGE_CURVE ( 'NONE', #57450, #88820, #46754, .T. ) ;
#84182=VERTEX_POINT ( 'NONE', #81326 ) ;
#84364=LINE ( 'NONE', #79218, #44352 ) ;
#84483=ORIENTED_EDGE ( 'NONE', *, *, #82743, .F. ) ;
#84498=EDGE_LOOP ( 'NONE', ( #18531, #59321, #81035, #26010 ) ) ;
#84692=DIRECTION ( 'NONE',  ( 0.000000000000000000, -0.000000000000000000, 1.000000000000000000 ) ) ;
#84745=CARTESIAN_POINT ( 'NONE',  ( 30.00000000000001776, 127.0000000000000000, 114.8826257785461280 ) ) ;
#84948=ORIENTED_EDGE ( 'NONE', *, *, #35969, .F. ) ;
#85031=CARTESIAN_POINT ( 'NONE',  ( 30.00000000000001776, 172.0000000000000000, 113.8826257785461280 ) ) ;
#85213=PLANE ( 'NONE',  #6549 ) ;
#85490=VECTOR ( 'NONE', #75474, 1000.000000000000000 ) ;
#85704=( GEOMETRIC_REPRESENTATION_CONTEXT ( 3 ) GLOBAL_UNCERTAINTY_ASSIGNED_CONTEXT ( ( #88101 ) ) GLOBAL_UNIT_ASSIGNED_CONTEXT ( ( #63280, #21966, #41471 ) ) REPRESENTATION_CONTEXT ( 'NONE', 'WORKASPACE' ) );
#85892=LINE ( 'NONE', #23663, #39970 ) ;
#86313=ORIENTED_EDGE ( 'NONE', *, *, #14732, .T. ) ;
#86361=DIRECTION ( 'NONE',  ( -1.000000000000000000, 0.000000000000000000, 2.973811673103097665E-16 ) ) ;
#86384=PLANE ( 'NONE',  #49407 ) ;
#86472=CARTESIAN_POINT ( 'NONE',  ( 0.000000000000000000, 172.0000000000000000, 0.000000000000000000 ) ) ;
#86622=ORIENTED_EDGE ( 'NONE', *, *, #86670, .F. ) ;
#86670=EDGE_CURVE ( 'NONE', #75853, #89067, #18011, .T. ) ;
#86830=DIRECTION ( 'NONE',  ( 0.000000000000000000, -1.000000000000000000, 0.000000000000000000 ) ) ;
#86996=CARTESIAN_POINT ( 'NONE',  ( 29.00000000000003553, 127.0000000000000000, 183.8826257785461280 ) ) ;
#87058=LINE ( 'NONE', #17124, #16735 ) ;
#87182=EDGE_CURVE ( 'NONE', #57450, #11953, #48, .T. ) ;
#88028=ADVANCED_FACE ( 'NONE', ( #32104 ), #59799, .F. ) ;
#88101=UNCERTAINTY_MEASURE_WITH_UNIT (LENGTH_MEASURE( 1.000000000000000082E-05 ), #63280, 'distance_accuracy_value', 'NONE');
#88249=CARTESIAN_POINT ( 'NONE',  ( -29.99999999999998224, 171.0000000000000000, 113.8826257785461280 ) ) ;
#88261=DIRECTION ( 'NONE',  ( 0.7071067811865489050, -0.7071067811865462405, 0.000000000000000000 ) ) ;
#88820=VERTEX_POINT ( 'NONE', #71906 ) ;
#89067=VERTEX_POINT ( 'NONE', #79918 ) ;
#89398=EDGE_CURVE ( 'NONE', #46473, #11953, #23641, .T. ) ;
#89409=PLANE ( 'NONE',  #17006 ) ;
#89443=VECTOR ( 'NONE', #35502, 1000.000000000000114 ) ;
#89572=DIRECTION ( 'NONE',  ( -2.973811673103097665E-16, 0.000000000000000000, -1.000000000000000000 ) ) ;
#89656=CARTESIAN_POINT ( 'NONE',  ( 0.000000000000000000, 0.000000000000000000, 0.000000000000000000 ) ) ;
#89895=PRODUCT_DEFINITION_CONTEXT ( 'detailed design', #23172, 'design' ) ;
ENDSEC;
END-ISO-10303-21;
